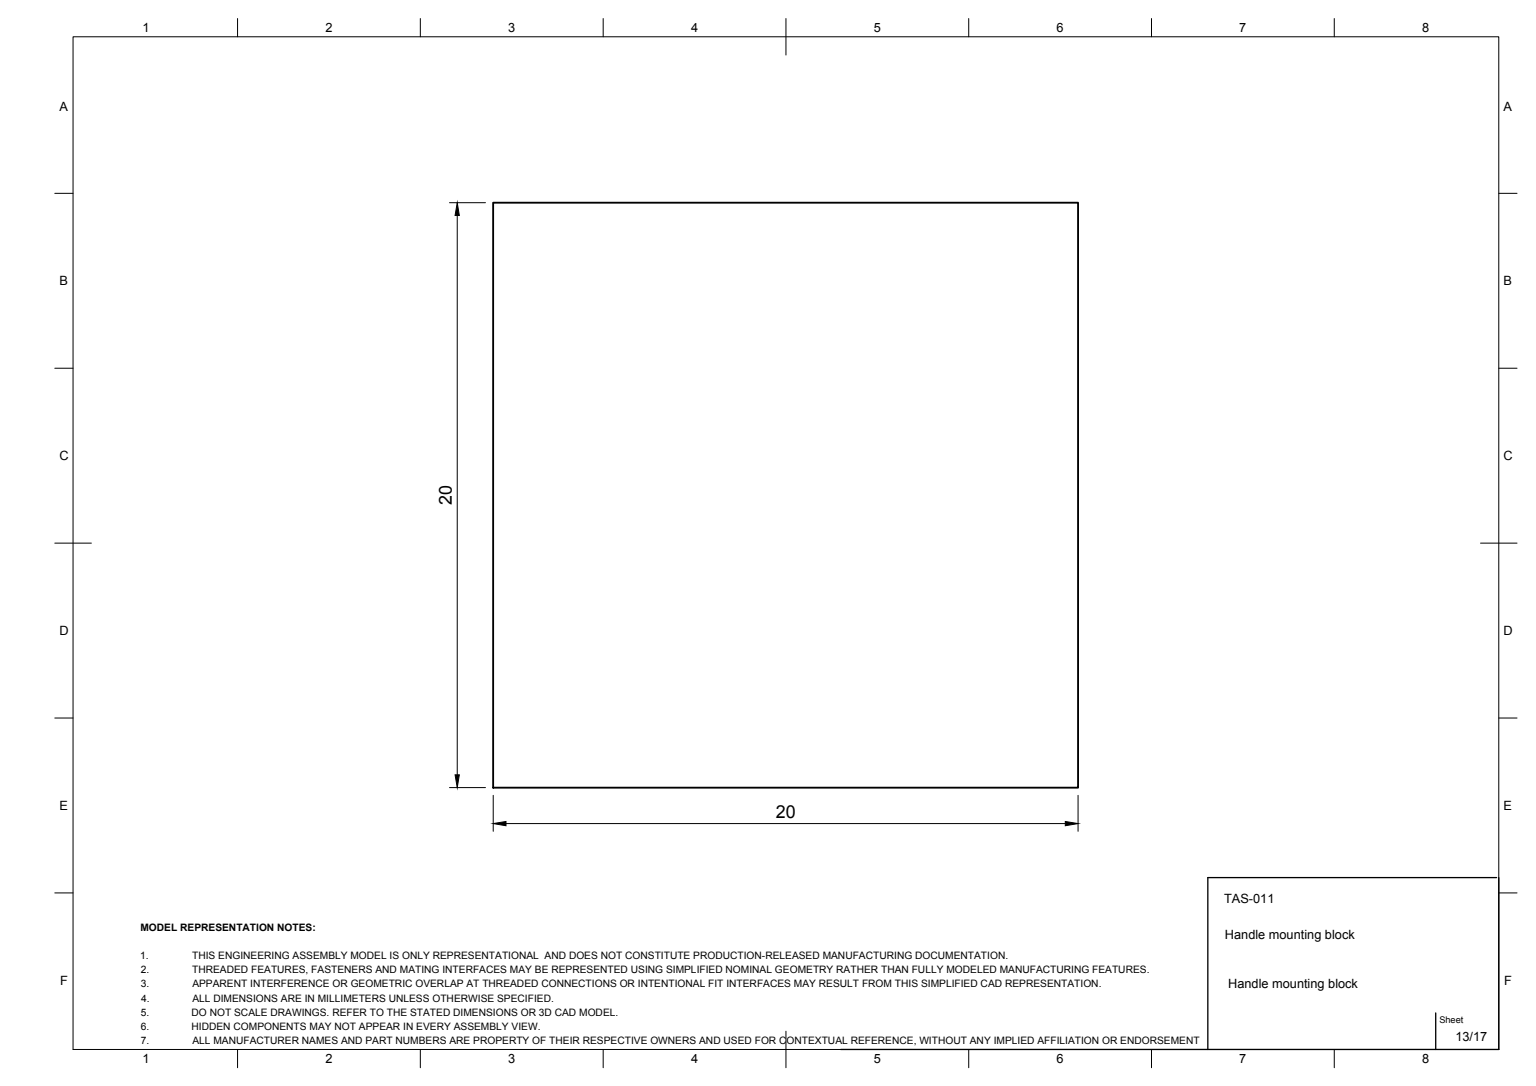
ISO-10303-21;
HEADER;
/* Generated by software containing ST-Developer
 * from STEP Tools, Inc. (www.steptools.com) 
 */

FILE_DESCRIPTION(
/* description */ (
'Independent manual bench leaf bending machine,200mm work width. Fabri
cated welded frame and folding leaf, repeated bushed and fully retaine
d hinge hardware, two handles with bonded grips, beveled clamping beam
 and modeledM12 clamp screws.2mm omitted-workpiece assembly reference 
gap, not a capacity claim. Native135deg hinge travel. Weld sizing, pro
duction fits, material condition, bending capacity, strength and life 
unassigned.'),
/* implementation_level */ '2;1');

FILE_NAME(
/* name */ 'Handle mounting block.step',
/* time_stamp */ '2026-11-14T09:11:34-08:00',
/* author */ (''),
/* organization */ (''),
/* preprocessor_version */ 'ST-DEVELOPER v20.2',
/* originating_system */ 'Autodesk Translation Framework v15.17.0.0',
/* authorisation */ '');

FILE_SCHEMA (('AUTOMOTIVE_DESIGN { 1 0 10303 214 3 1 1 }'));
ENDSEC;

DATA;
#10=MECHANICAL_DESIGN_GEOMETRIC_PRESENTATION_REPRESENTATION('',(#458),#37701);
#422=SHAPE_REPRESENTATION_RELATIONSHIP('SRR','None',#37791,#440);
#440=ADVANCED_BREP_SHAPE_REPRESENTATION('',(#476),#37695);
#458=STYLED_ITEM('',(#37879),#476);
#476=MANIFOLD_SOLID_BREP('Body1',#4156);
#580=PLANE('',#4613);
#581=PLANE('',#4614);
#582=PLANE('',#4615);
#583=PLANE('',#4616);
#584=PLANE('',#4617);
#585=PLANE('',#4618);
#781=FACE_OUTER_BOUND('',#1021,.T.);
#782=FACE_OUTER_BOUND('',#1022,.T.);
#783=FACE_OUTER_BOUND('',#1023,.T.);
#784=FACE_OUTER_BOUND('',#1024,.T.);
#785=FACE_OUTER_BOUND('',#1025,.T.);
#786=FACE_OUTER_BOUND('',#1026,.T.);
#1021=EDGE_LOOP('',(#3709,#3710,#3711,#3712));
#1022=EDGE_LOOP('',(#3713,#3714,#3715,#3716));
#1023=EDGE_LOOP('',(#3717,#3718,#3719,#3720));
#1024=EDGE_LOOP('',(#3721,#3722,#3723,#3724));
#1025=EDGE_LOOP('',(#3725,#3726,#3727,#3728));
#1026=EDGE_LOOP('',(#3729,#3730,#3731,#3732));
#1280=LINE('',#37508,#1529);
#1281=LINE('',#37510,#1530);
#1282=LINE('',#37512,#1531);
#1283=LINE('',#37513,#1532);
#1284=LINE('',#37516,#1533);
#1285=LINE('',#37518,#1534);
#1286=LINE('',#37519,#1535);
#1287=LINE('',#37522,#1536);
#1288=LINE('',#37524,#1537);
#1289=LINE('',#37525,#1538);
#1290=LINE('',#37527,#1539);
#1291=LINE('',#37528,#1540);
#1529=VECTOR('',#5433,10.);
#1530=VECTOR('',#5434,10.);
#1531=VECTOR('',#5435,10.);
#1532=VECTOR('',#5436,10.);
#1533=VECTOR('',#5439,10.);
#1534=VECTOR('',#5440,10.);
#1535=VECTOR('',#5441,10.);
#1536=VECTOR('',#5444,10.);
#1537=VECTOR('',#5445,10.);
#1538=VECTOR('',#5446,10.);
#1539=VECTOR('',#5449,10.);
#1540=VECTOR('',#5450,10.);
#2019=VERTEX_POINT('',#37506);
#2020=VERTEX_POINT('',#37507);
#2021=VERTEX_POINT('',#37509);
#2022=VERTEX_POINT('',#37511);
#2023=VERTEX_POINT('',#37515);
#2024=VERTEX_POINT('',#37517);
#2025=VERTEX_POINT('',#37521);
#2026=VERTEX_POINT('',#37523);
#2588=EDGE_CURVE('',#2019,#2020,#1280,.T.);
#2589=EDGE_CURVE('',#2020,#2021,#1281,.T.);
#2590=EDGE_CURVE('',#2022,#2021,#1282,.T.);
#2591=EDGE_CURVE('',#2019,#2022,#1283,.T.);
#2592=EDGE_CURVE('',#2023,#2019,#1284,.T.);
#2593=EDGE_CURVE('',#2024,#2022,#1285,.T.);
#2594=EDGE_CURVE('',#2023,#2024,#1286,.T.);
#2595=EDGE_CURVE('',#2025,#2023,#1287,.T.);
#2596=EDGE_CURVE('',#2026,#2024,#1288,.T.);
#2597=EDGE_CURVE('',#2025,#2026,#1289,.T.);
#2598=EDGE_CURVE('',#2020,#2025,#1290,.T.);
#2599=EDGE_CURVE('',#2021,#2026,#1291,.T.);
#3709=ORIENTED_EDGE('',*,*,#2588,.T.);
#3710=ORIENTED_EDGE('',*,*,#2589,.T.);
#3711=ORIENTED_EDGE('',*,*,#2590,.F.);
#3712=ORIENTED_EDGE('',*,*,#2591,.F.);
#3713=ORIENTED_EDGE('',*,*,#2592,.T.);
#3714=ORIENTED_EDGE('',*,*,#2591,.T.);
#3715=ORIENTED_EDGE('',*,*,#2593,.F.);
#3716=ORIENTED_EDGE('',*,*,#2594,.F.);
#3717=ORIENTED_EDGE('',*,*,#2595,.T.);
#3718=ORIENTED_EDGE('',*,*,#2594,.T.);
#3719=ORIENTED_EDGE('',*,*,#2596,.F.);
#3720=ORIENTED_EDGE('',*,*,#2597,.F.);
#3721=ORIENTED_EDGE('',*,*,#2598,.T.);
#3722=ORIENTED_EDGE('',*,*,#2597,.T.);
#3723=ORIENTED_EDGE('',*,*,#2599,.F.);
#3724=ORIENTED_EDGE('',*,*,#2589,.F.);
#3725=ORIENTED_EDGE('',*,*,#2599,.T.);
#3726=ORIENTED_EDGE('',*,*,#2596,.T.);
#3727=ORIENTED_EDGE('',*,*,#2593,.T.);
#3728=ORIENTED_EDGE('',*,*,#2590,.T.);
#3729=ORIENTED_EDGE('',*,*,#2598,.F.);
#3730=ORIENTED_EDGE('',*,*,#2588,.F.);
#3731=ORIENTED_EDGE('',*,*,#2592,.F.);
#3732=ORIENTED_EDGE('',*,*,#2595,.F.);
#4111=ADVANCED_FACE('',(#781),#580,.T.);
#4112=ADVANCED_FACE('',(#782),#581,.T.);
#4113=ADVANCED_FACE('',(#783),#582,.T.);
#4114=ADVANCED_FACE('',(#784),#583,.T.);
#4115=ADVANCED_FACE('',(#785),#584,.T.);
#4116=ADVANCED_FACE('',(#786),#585,.F.);
#4156=CLOSED_SHELL('',(#4111,#4112,#4113,#4114,#4115,#4116));
#4612=AXIS2_PLACEMENT_3D('',#37504,#5429,#5430);
#4613=AXIS2_PLACEMENT_3D('',#37505,#5431,#5432);
#4614=AXIS2_PLACEMENT_3D('',#37514,#5437,#5438);
#4615=AXIS2_PLACEMENT_3D('',#37520,#5442,#5443);
#4616=AXIS2_PLACEMENT_3D('',#37526,#5447,#5448);
#4617=AXIS2_PLACEMENT_3D('',#37529,#5451,#5452);
#4618=AXIS2_PLACEMENT_3D('',#37530,#5453,#5454);
#5429=DIRECTION('axis',(0.,0.,1.));
#5430=DIRECTION('refdir',(1.,0.,0.));
#5431=DIRECTION('center_axis',(0.,1.,0.));
#5432=DIRECTION('ref_axis',(-1.,0.,0.));
#5433=DIRECTION('',(-1.,0.,0.));
#5434=DIRECTION('',(0.,0.,1.));
#5435=DIRECTION('',(-1.,0.,0.));
#5436=DIRECTION('',(0.,0.,1.));
#5437=DIRECTION('center_axis',(1.,0.,0.));
#5438=DIRECTION('ref_axis',(0.,1.,0.));
#5439=DIRECTION('',(0.,1.,0.));
#5440=DIRECTION('',(0.,1.,0.));
#5441=DIRECTION('',(0.,0.,1.));
#5442=DIRECTION('center_axis',(0.,-1.,0.));
#5443=DIRECTION('ref_axis',(1.,0.,0.));
#5444=DIRECTION('',(1.,0.,0.));
#5445=DIRECTION('',(1.,0.,0.));
#5446=DIRECTION('',(0.,0.,1.));
#5447=DIRECTION('center_axis',(-1.,0.,0.));
#5448=DIRECTION('ref_axis',(0.,-1.,0.));
#5449=DIRECTION('',(0.,-1.,0.));
#5450=DIRECTION('',(0.,-1.,0.));
#5451=DIRECTION('center_axis',(0.,0.,1.));
#5452=DIRECTION('ref_axis',(1.,0.,0.));
#5453=DIRECTION('center_axis',(0.,0.,1.));
#5454=DIRECTION('ref_axis',(1.,0.,0.));
#37504=CARTESIAN_POINT('',(0.,0.,0.));
#37505=CARTESIAN_POINT('Origin',(70.,10.,10.));
#37506=CARTESIAN_POINT('',(70.,10.,10.));
#37507=CARTESIAN_POINT('',(50.,10.,10.));
#37508=CARTESIAN_POINT('',(70.,10.,10.));
#37509=CARTESIAN_POINT('',(50.,10.,30.));
#37510=CARTESIAN_POINT('',(50.,10.,10.));
#37511=CARTESIAN_POINT('',(70.,10.,30.));
#37512=CARTESIAN_POINT('',(70.,10.,30.));
#37513=CARTESIAN_POINT('',(70.,10.,10.));
#37514=CARTESIAN_POINT('Origin',(70.,-10.,10.));
#37515=CARTESIAN_POINT('',(70.,-10.,10.));
#37516=CARTESIAN_POINT('',(70.,-10.,10.));
#37517=CARTESIAN_POINT('',(70.,-10.,30.));
#37518=CARTESIAN_POINT('',(70.,-10.,30.));
#37519=CARTESIAN_POINT('',(70.,-10.,10.));
#37520=CARTESIAN_POINT('Origin',(50.,-10.,10.));
#37521=CARTESIAN_POINT('',(50.,-10.,10.));
#37522=CARTESIAN_POINT('',(50.,-10.,10.));
#37523=CARTESIAN_POINT('',(50.,-10.,30.));
#37524=CARTESIAN_POINT('',(50.,-10.,30.));
#37525=CARTESIAN_POINT('',(50.,-10.,10.));
#37526=CARTESIAN_POINT('Origin',(50.,10.,10.));
#37527=CARTESIAN_POINT('',(50.,10.,10.));
#37528=CARTESIAN_POINT('',(50.,10.,30.));
#37529=CARTESIAN_POINT('Origin',(60.,0.,30.));
#37530=CARTESIAN_POINT('Origin',(60.,0.,10.));
#37675=UNCERTAINTY_MEASURE_WITH_UNIT(LENGTH_MEASURE(0.01),#37702,
'DISTANCE_ACCURACY_VALUE',
'Maximum model space distance between geometric entities at asserted c
onnectivities');
#37681=UNCERTAINTY_MEASURE_WITH_UNIT(LENGTH_MEASURE(0.01),#37702,
'DISTANCE_ACCURACY_VALUE',
'Maximum model space distance between geometric entities at asserted c
onnectivities');
#37695=(
GEOMETRIC_REPRESENTATION_CONTEXT(3)
GLOBAL_UNCERTAINTY_ASSIGNED_CONTEXT((#37675))
GLOBAL_UNIT_ASSIGNED_CONTEXT((#37702,#37704,#37705))
REPRESENTATION_CONTEXT('','3D')
);
#37701=(
GEOMETRIC_REPRESENTATION_CONTEXT(3)
GLOBAL_UNCERTAINTY_ASSIGNED_CONTEXT((#37681))
GLOBAL_UNIT_ASSIGNED_CONTEXT((#37702,#37704,#37705))
REPRESENTATION_CONTEXT('','3D')
);
#37702=(
LENGTH_UNIT()
NAMED_UNIT(*)
SI_UNIT(.MILLI.,.METRE.)
);
#37704=(
NAMED_UNIT(*)
PLANE_ANGLE_UNIT()
SI_UNIT($,.RADIAN.)
);
#37705=(
NAMED_UNIT(*)
SI_UNIT($,.STERADIAN.)
SOLID_ANGLE_UNIT()
);
#37719=SHAPE_DEFINITION_REPRESENTATION(#37738,#37791);
#37738=PRODUCT_DEFINITION_SHAPE('',$,#37811);
#37791=SHAPE_REPRESENTATION('',(#4612),#37695);
#37797=PRODUCT_DEFINITION_CONTEXT('part definition',#37856,'design');
#37811=PRODUCT_DEFINITION('Handle mounting block',
'Handle mounting block',#37830,#37797);
#37830=PRODUCT_DEFINITION_FORMATION('',$,#37871);
#37856=APPLICATION_CONTEXT(
'Core Data for Automotive Mechanical Design Process');
#37857=PRODUCT_CONTEXT('part definition',#37856,'mechanical');
#37871=PRODUCT('Handle mounting block','Handle mounting block',$,(#37857));
#37879=PRESENTATION_STYLE_ASSIGNMENT((#37887));
#37887=SURFACE_STYLE_USAGE(.BOTH.,#37895);
#37895=SURFACE_SIDE_STYLE('',(#37903));
#37903=SURFACE_STYLE_FILL_AREA(#37911);
#37911=FILL_AREA_STYLE('Opaque(104,114,127)',(#37919));
#37919=FILL_AREA_STYLE_COLOUR('Opaque(104,114,127)',#37927);
#37927=COLOUR_RGB('Opaque(104,114,127)',0.407843137254902,0.447058823529412,
0.498039215686275);
ENDSEC;
END-ISO-10303-21;
